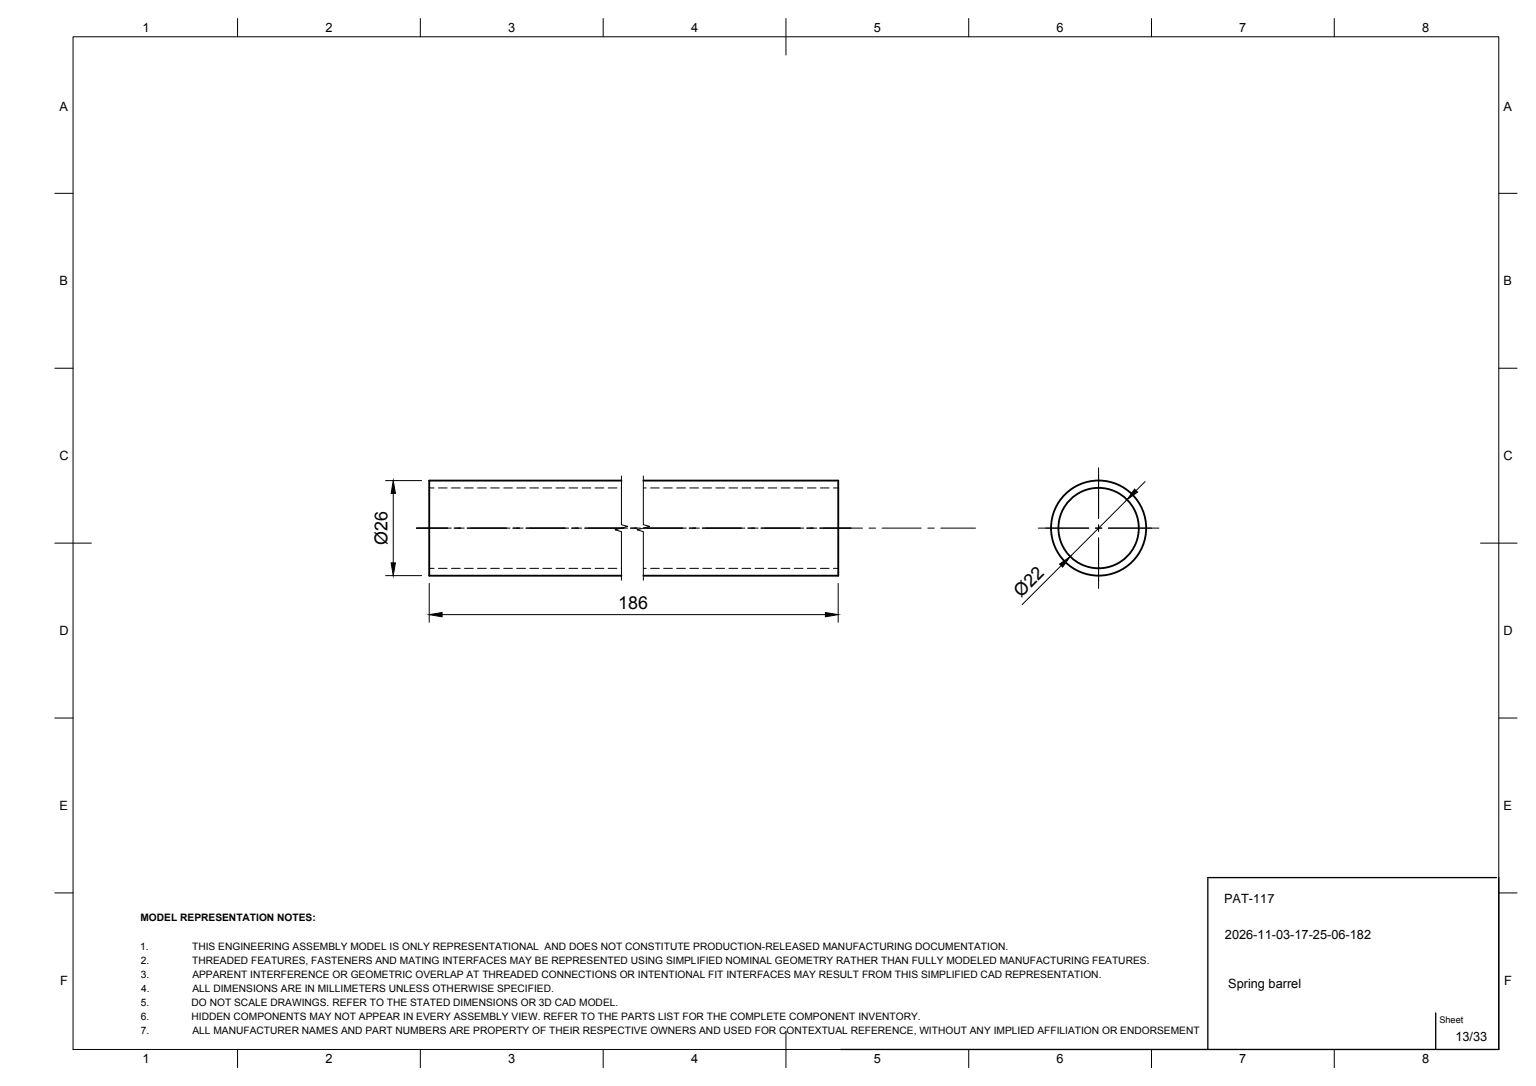
ISO-10303-21;
HEADER;
/* Generated by software containing ST-Developer
 * from STEP Tools, Inc. (www.steptools.com) 
 */

FILE_DESCRIPTION(
/* description */ ('Counterbalanced vertical column'),
/* implementation_level */ '2;1');

FILE_NAME(
/* name */ 'Spring barrel.step',
/* time_stamp */ '2026-10-29T16:47:22-07:00',
/* author */ (''),
/* organization */ (''),
/* preprocessor_version */ 'ST-DEVELOPER v20.2',
/* originating_system */ 'Autodesk Translation Framework v15.17.0.0',
/* authorisation */ '');

FILE_SCHEMA (('AUTOMOTIVE_DESIGN { 1 0 10303 214 3 1 1 }'));
ENDSEC;

DATA;
#10=MECHANICAL_DESIGN_GEOMETRIC_PRESENTATION_REPRESENTATION('',(#358),#15040);
#288=SHAPE_REPRESENTATION_RELATIONSHIP('SRR','None',#15192,#323);
#323=ADVANCED_BREP_SHAPE_REPRESENTATION('',(#393),#15011);
#358=STYLED_ITEM('',(#15457),#393);
#393=MANIFOLD_SOLID_BREP('Body1',#7081);
#450=FACE_BOUND('',#1343,.T.);
#451=FACE_BOUND('',#1345,.T.);
#585=PLANE('',#7632);
#586=PLANE('',#7633);
#901=FACE_OUTER_BOUND('',#1340,.T.);
#902=FACE_OUTER_BOUND('',#1341,.T.);
#903=FACE_OUTER_BOUND('',#1342,.T.);
#904=FACE_OUTER_BOUND('',#1344,.T.);
#1340=EDGE_LOOP('',(#5106,#5107,#5108,#5109));
#1341=EDGE_LOOP('',(#5110,#5111,#5112,#5113));
#1342=EDGE_LOOP('',(#5114));
#1343=EDGE_LOOP('',(#5115));
#1344=EDGE_LOOP('',(#5116));
#1345=EDGE_LOOP('',(#5117));
#1868=LINE('',#10693,#2539);
#1869=LINE('',#10699,#2540);
#2539=VECTOR('',#8598,1.1);
#2540=VECTOR('',#8605,1.3);
#3135=CIRCLE('',#7627,1.1);
#3136=CIRCLE('',#7628,1.1);
#3137=CIRCLE('',#7630,1.3);
#3138=CIRCLE('',#7631,1.3);
#3412=VERTEX_POINT('',#10690);
#3413=VERTEX_POINT('',#10692);
#3414=VERTEX_POINT('',#10696);
#3415=VERTEX_POINT('',#10698);
#4054=EDGE_CURVE('',#3412,#3412,#3135,.T.);
#4055=EDGE_CURVE('',#3412,#3413,#1868,.T.);
#4056=EDGE_CURVE('',#3413,#3413,#3136,.T.);
#4057=EDGE_CURVE('',#3414,#3414,#3137,.T.);
#4058=EDGE_CURVE('',#3414,#3415,#1869,.T.);
#4059=EDGE_CURVE('',#3415,#3415,#3138,.T.);
#5106=ORIENTED_EDGE('',*,*,#4054,.F.);
#5107=ORIENTED_EDGE('',*,*,#4055,.T.);
#5108=ORIENTED_EDGE('',*,*,#4056,.T.);
#5109=ORIENTED_EDGE('',*,*,#4055,.F.);
#5110=ORIENTED_EDGE('',*,*,#4057,.F.);
#5111=ORIENTED_EDGE('',*,*,#4058,.T.);
#5112=ORIENTED_EDGE('',*,*,#4059,.T.);
#5113=ORIENTED_EDGE('',*,*,#4058,.F.);
#5114=ORIENTED_EDGE('',*,*,#4057,.T.);
#5115=ORIENTED_EDGE('',*,*,#4054,.T.);
#5116=ORIENTED_EDGE('',*,*,#4059,.F.);
#5117=ORIENTED_EDGE('',*,*,#4056,.F.);
#6595=CYLINDRICAL_SURFACE('',#7626,1.1);
#6596=CYLINDRICAL_SURFACE('',#7629,1.3);
#6743=ADVANCED_FACE('',(#901),#6595,.F.);
#6744=ADVANCED_FACE('',(#902),#6596,.T.);
#6745=ADVANCED_FACE('',(#903,#450),#585,.T.);
#6746=ADVANCED_FACE('',(#904,#451),#586,.F.);
#7081=CLOSED_SHELL('',(#6743,#6744,#6745,#6746));
#7625=AXIS2_PLACEMENT_3D('',#10688,#8592,#8593);
#7626=AXIS2_PLACEMENT_3D('',#10689,#8594,#8595);
#7627=AXIS2_PLACEMENT_3D('',#10691,#8596,#8597);
#7628=AXIS2_PLACEMENT_3D('',#10694,#8599,#8600);
#7629=AXIS2_PLACEMENT_3D('',#10695,#8601,#8602);
#7630=AXIS2_PLACEMENT_3D('',#10697,#8603,#8604);
#7631=AXIS2_PLACEMENT_3D('',#10700,#8606,#8607);
#7632=AXIS2_PLACEMENT_3D('',#10701,#8608,#8609);
#7633=AXIS2_PLACEMENT_3D('',#10702,#8610,#8611);
#8592=DIRECTION('axis',(0.,0.,1.));
#8593=DIRECTION('refdir',(1.,0.,0.));
#8594=DIRECTION('center_axis',(0.,0.,1.));
#8595=DIRECTION('ref_axis',(1.,0.,0.));
#8596=DIRECTION('center_axis',(0.,0.,-1.));
#8597=DIRECTION('ref_axis',(1.,0.,0.));
#8598=DIRECTION('',(0.,0.,-1.));
#8599=DIRECTION('center_axis',(0.,0.,-1.));
#8600=DIRECTION('ref_axis',(1.,0.,0.));
#8601=DIRECTION('center_axis',(0.,0.,1.));
#8602=DIRECTION('ref_axis',(1.,0.,0.));
#8603=DIRECTION('center_axis',(0.,0.,1.));
#8604=DIRECTION('ref_axis',(1.,0.,0.));
#8605=DIRECTION('',(0.,0.,-1.));
#8606=DIRECTION('center_axis',(0.,0.,1.));
#8607=DIRECTION('ref_axis',(1.,0.,0.));
#8608=DIRECTION('center_axis',(0.,0.,1.));
#8609=DIRECTION('ref_axis',(1.,0.,0.));
#8610=DIRECTION('center_axis',(0.,0.,1.));
#8611=DIRECTION('ref_axis',(1.,0.,0.));
#10688=CARTESIAN_POINT('',(0.,0.,0.));
#10689=CARTESIAN_POINT('Origin',(-7.,0.,1.4));
#10690=CARTESIAN_POINT('',(-8.1,-1.34711147906209E-16,20.));
#10691=CARTESIAN_POINT('Origin',(-7.,0.,20.));
#10692=CARTESIAN_POINT('',(-8.1,-1.34711147906209E-16,1.4));
#10693=CARTESIAN_POINT('',(-8.1,-1.34711147906209E-16,1.4));
#10694=CARTESIAN_POINT('Origin',(-7.,0.,1.4));
#10695=CARTESIAN_POINT('Origin',(-7.,0.,1.4));
#10696=CARTESIAN_POINT('',(-8.3,-1.59204083889156E-16,20.));
#10697=CARTESIAN_POINT('Origin',(-7.,0.,20.));
#10698=CARTESIAN_POINT('',(-8.3,-1.59204083889156E-16,1.4));
#10699=CARTESIAN_POINT('',(-8.3,-1.59204083889156E-16,1.4));
#10700=CARTESIAN_POINT('Origin',(-7.,0.,1.4));
#10701=CARTESIAN_POINT('Origin',(-7.,0.,20.));
#10702=CARTESIAN_POINT('Origin',(-7.,0.,1.4));
#14971=UNCERTAINTY_MEASURE_WITH_UNIT(LENGTH_MEASURE(0.001),#15041,
'DISTANCE_ACCURACY_VALUE',
'Maximum model space distance between geometric entities at asserted c
onnectivities');
#15000=UNCERTAINTY_MEASURE_WITH_UNIT(LENGTH_MEASURE(0.001),#15041,
'DISTANCE_ACCURACY_VALUE',
'Maximum model space distance between geometric entities at asserted c
onnectivities');
#15011=(
GEOMETRIC_REPRESENTATION_CONTEXT(3)
GLOBAL_UNCERTAINTY_ASSIGNED_CONTEXT((#14971))
GLOBAL_UNIT_ASSIGNED_CONTEXT((#15041,#15043,#15044))
REPRESENTATION_CONTEXT('','3D')
);
#15040=(
GEOMETRIC_REPRESENTATION_CONTEXT(3)
GLOBAL_UNCERTAINTY_ASSIGNED_CONTEXT((#15000))
GLOBAL_UNIT_ASSIGNED_CONTEXT((#15041,#15043,#15044))
REPRESENTATION_CONTEXT('','3D')
);
#15041=(
LENGTH_UNIT()
NAMED_UNIT(*)
SI_UNIT(.CENTI.,.METRE.)
);
#15043=(
NAMED_UNIT(*)
PLANE_ANGLE_UNIT()
SI_UNIT($,.RADIAN.)
);
#15044=(
NAMED_UNIT(*)
SI_UNIT($,.STERADIAN.)
SOLID_ANGLE_UNIT()
);
#15055=SHAPE_DEFINITION_REPRESENTATION(#15094,#15192);
#15094=PRODUCT_DEFINITION_SHAPE('',$,#15232);
#15192=SHAPE_REPRESENTATION('',(#7625),#15011);
#15221=PRODUCT_DEFINITION_CONTEXT('part definition',#15340,'design');
#15232=PRODUCT_DEFINITION('Spring barrel','Spring barrel',#15271,#15221);
#15271=PRODUCT_DEFINITION_FORMATION('',$,#15352);
#15340=APPLICATION_CONTEXT(
'Core Data for Automotive Mechanical Design Process');
#15341=PRODUCT_CONTEXT('part definition',#15340,'mechanical');
#15352=PRODUCT('Spring barrel','Spring barrel','Spring barrel',(#15341));
#15451=COLOUR_RGB('Grey',0.48,0.52,0.57);
#15452=FILL_AREA_STYLE_COLOUR('',#15451);
#15453=FILL_AREA_STYLE('',(#15452));
#15454=SURFACE_STYLE_FILL_AREA(#15453);
#15455=SURFACE_SIDE_STYLE('',(#15454));
#15456=SURFACE_STYLE_USAGE(.BOTH.,#15455);
#15457=PRESENTATION_STYLE_ASSIGNMENT((#15456));
ENDSEC;
END-ISO-10303-21;
